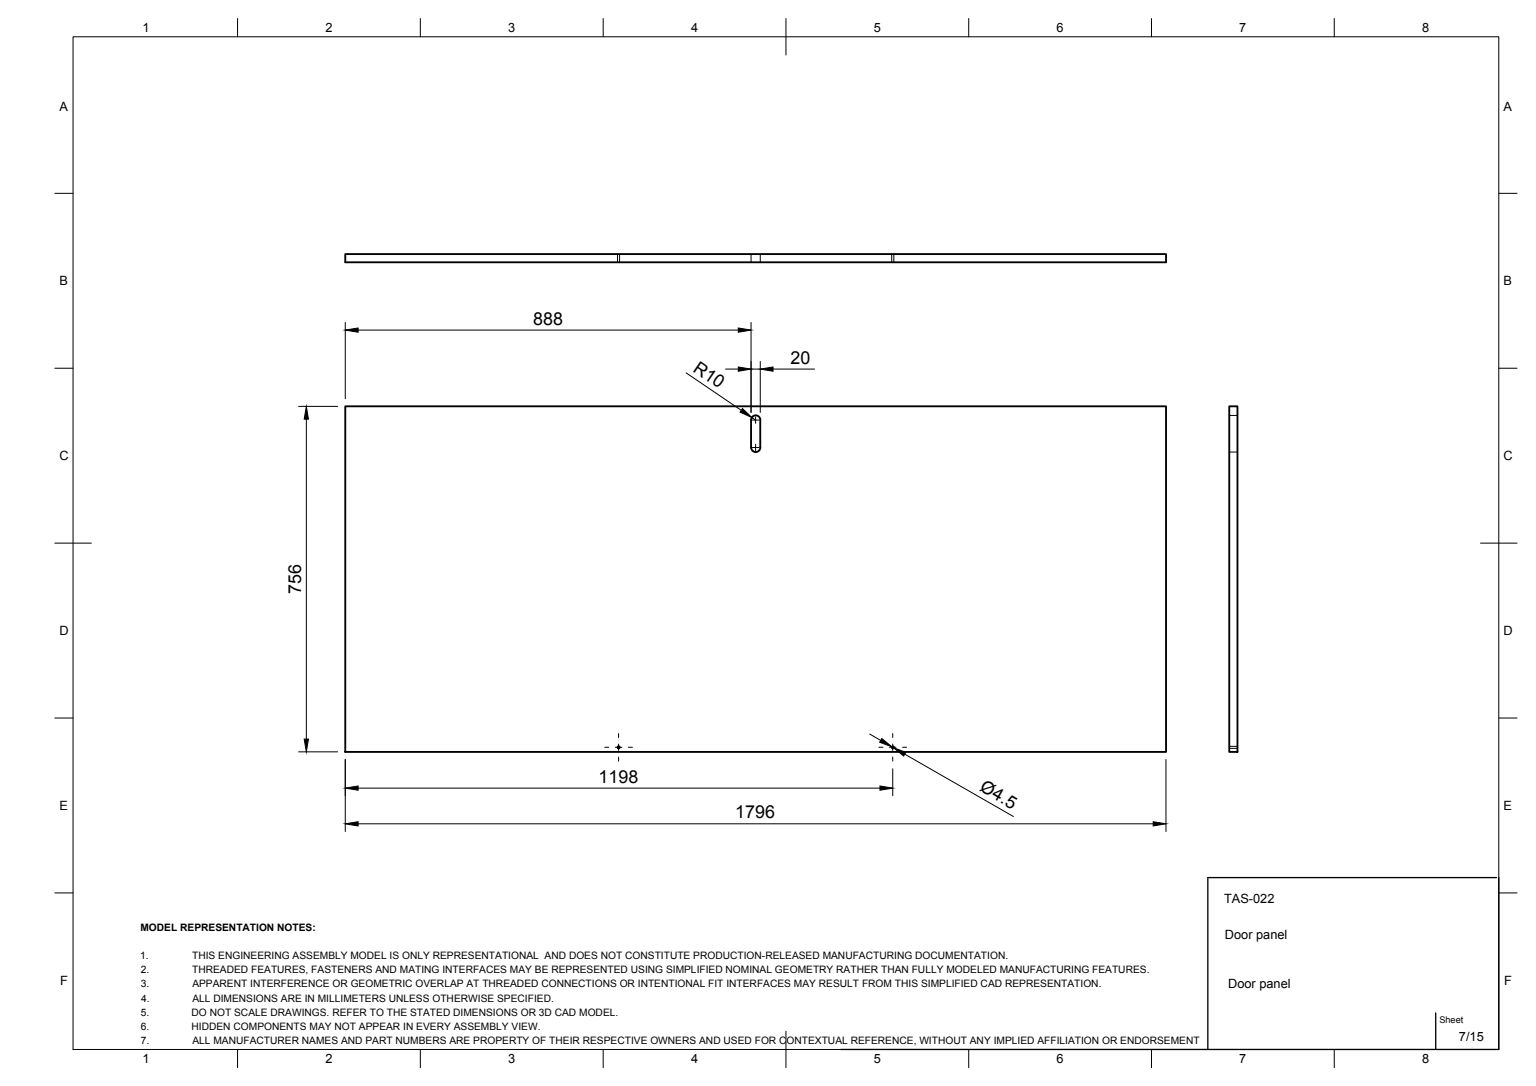
ISO-10303-21;
HEADER;
/* Generated by software containing ST-Developer
 * from STEP Tools, Inc. (www.steptools.com) 
 */

FILE_DESCRIPTION(
/* description */ (''),
/* implementation_level */ '2;1');

FILE_NAME(
/* name */ 'Door panel.step',
/* time_stamp */ '2026-11-15T21:02:08-08:00',
/* author */ (''),
/* organization */ (''),
/* preprocessor_version */ 'ST-DEVELOPER v20.2',
/* originating_system */ 'Autodesk Translation Framework v15.17.0.0',
/* authorisation */ '');

FILE_SCHEMA (('AUTOMOTIVE_DESIGN { 1 0 10303 214 3 1 1 }'));
ENDSEC;

DATA;
#10=MECHANICAL_DESIGN_GEOMETRIC_PRESENTATION_REPRESENTATION('',(#603),#31566);
#381=FACE_BOUND('',#914,.T.);
#382=FACE_BOUND('',#915,.T.);
#383=FACE_BOUND('',#916,.T.);
#384=FACE_BOUND('',#919,.T.);
#385=FACE_BOUND('',#920,.T.);
#386=FACE_BOUND('',#921,.T.);
#417=CIRCLE('',#5907,1.);
#418=CIRCLE('',#5908,1.);
#419=CIRCLE('',#5911,1.);
#420=CIRCLE('',#5912,1.);
#421=CIRCLE('',#5914,0.225);
#422=CIRCLE('',#5915,0.225);
#423=CIRCLE('',#5917,0.225);
#424=CIRCLE('',#5918,0.225);
#490=CYLINDRICAL_SURFACE('',#5906,1.);
#491=CYLINDRICAL_SURFACE('',#5910,1.);
#492=CYLINDRICAL_SURFACE('',#5913,0.225);
#493=CYLINDRICAL_SURFACE('',#5916,0.225);
#573=SHAPE_REPRESENTATION_RELATIONSHIP('SRR','None',#31637,#588);
#588=ADVANCED_BREP_SHAPE_REPRESENTATION('',(#618),#31552);
#603=STYLED_ITEM('',(#31721),#618);
#618=MANIFOLD_SOLID_BREP('Body1',#5716);
#638=FACE_OUTER_BOUND('',#907,.T.);
#639=FACE_OUTER_BOUND('',#908,.T.);
#640=FACE_OUTER_BOUND('',#909,.T.);
#641=FACE_OUTER_BOUND('',#910,.T.);
#642=FACE_OUTER_BOUND('',#911,.T.);
#643=FACE_OUTER_BOUND('',#912,.T.);
#644=FACE_OUTER_BOUND('',#913,.T.);
#645=FACE_OUTER_BOUND('',#917,.T.);
#646=FACE_OUTER_BOUND('',#918,.T.);
#647=FACE_OUTER_BOUND('',#922,.T.);
#648=FACE_OUTER_BOUND('',#923,.T.);
#649=FACE_OUTER_BOUND('',#924,.T.);
#907=EDGE_LOOP('',(#3651,#3652,#3653,#3654));
#908=EDGE_LOOP('',(#3655,#3656,#3657,#3658));
#909=EDGE_LOOP('',(#3659,#3660,#3661,#3662));
#910=EDGE_LOOP('',(#3663,#3664,#3665,#3666));
#911=EDGE_LOOP('',(#3667,#3668,#3669,#3670));
#912=EDGE_LOOP('',(#3671,#3672,#3673,#3674));
#913=EDGE_LOOP('',(#3675,#3676,#3677,#3678));
#914=EDGE_LOOP('',(#3679,#3680,#3681,#3682));
#915=EDGE_LOOP('',(#3683));
#916=EDGE_LOOP('',(#3684));
#917=EDGE_LOOP('',(#3685,#3686,#3687,#3688));
#918=EDGE_LOOP('',(#3689,#3690,#3691,#3692));
#919=EDGE_LOOP('',(#3693,#3694,#3695,#3696));
#920=EDGE_LOOP('',(#3697));
#921=EDGE_LOOP('',(#3698));
#922=EDGE_LOOP('',(#3699,#3700,#3701,#3702));
#923=EDGE_LOOP('',(#3703,#3704,#3705,#3706));
#924=EDGE_LOOP('',(#3707,#3708,#3709,#3710));
#1218=LINE('',#7593,#1725);
#1219=LINE('',#7595,#1726);
#1220=LINE('',#7597,#1727);
#1221=LINE('',#7598,#1728);
#1222=LINE('',#7603,#1729);
#1223=LINE('',#7607,#1730);
#1224=LINE('',#7609,#1731);
#1225=LINE('',#7610,#1732);
#1226=LINE('',#7618,#1733);
#1227=LINE('',#7624,#1734);
#1228=LINE('',#7629,#1735);
#1229=LINE('',#7631,#1736);
#1230=LINE('',#7633,#1737);
#1231=LINE('',#7634,#1738);
#1232=LINE('',#7637,#1739);
#1233=LINE('',#7639,#1740);
#1234=LINE('',#7640,#1741);
#1235=LINE('',#7643,#1742);
#1236=LINE('',#7645,#1743);
#1237=LINE('',#7646,#1744);
#1238=LINE('',#7648,#1745);
#1239=LINE('',#7649,#1746);
#1725=VECTOR('',#6314,1.);
#1726=VECTOR('',#6315,1.);
#1727=VECTOR('',#6316,1.);
#1728=VECTOR('',#6317,1.);
#1729=VECTOR('',#6322,1.);
#1730=VECTOR('',#6327,1.);
#1731=VECTOR('',#6328,1.);
#1732=VECTOR('',#6329,1.);
#1733=VECTOR('',#6340,0.225);
#1734=VECTOR('',#6347,0.225);
#1735=VECTOR('',#6352,1.);
#1736=VECTOR('',#6353,1.);
#1737=VECTOR('',#6354,1.);
#1738=VECTOR('',#6355,1.);
#1739=VECTOR('',#6358,1.);
#1740=VECTOR('',#6359,1.);
#1741=VECTOR('',#6360,1.);
#1742=VECTOR('',#6363,1.);
#1743=VECTOR('',#6364,1.);
#1744=VECTOR('',#6365,1.);
#1745=VECTOR('',#6368,1.);
#1746=VECTOR('',#6369,1.);
#2228=VERTEX_POINT('',#7591);
#2229=VERTEX_POINT('',#7592);
#2230=VERTEX_POINT('',#7594);
#2231=VERTEX_POINT('',#7596);
#2232=VERTEX_POINT('',#7600);
#2233=VERTEX_POINT('',#7602);
#2234=VERTEX_POINT('',#7606);
#2235=VERTEX_POINT('',#7608);
#2236=VERTEX_POINT('',#7615);
#2237=VERTEX_POINT('',#7617);
#2238=VERTEX_POINT('',#7621);
#2239=VERTEX_POINT('',#7623);
#2240=VERTEX_POINT('',#7627);
#2241=VERTEX_POINT('',#7628);
#2242=VERTEX_POINT('',#7630);
#2243=VERTEX_POINT('',#7632);
#2244=VERTEX_POINT('',#7636);
#2245=VERTEX_POINT('',#7638);
#2246=VERTEX_POINT('',#7642);
#2247=VERTEX_POINT('',#7644);
#2821=EDGE_CURVE('',#2228,#2229,#1218,.T.);
#2822=EDGE_CURVE('',#2228,#2230,#1219,.T.);
#2823=EDGE_CURVE('',#2231,#2230,#1220,.T.);
#2824=EDGE_CURVE('',#2229,#2231,#1221,.T.);
#2825=EDGE_CURVE('',#2232,#2228,#417,.T.);
#2826=EDGE_CURVE('',#2232,#2233,#1222,.T.);
#2827=EDGE_CURVE('',#2230,#2233,#418,.T.);
#2828=EDGE_CURVE('',#2234,#2232,#1223,.T.);
#2829=EDGE_CURVE('',#2234,#2235,#1224,.T.);
#2830=EDGE_CURVE('',#2233,#2235,#1225,.T.);
#2831=EDGE_CURVE('',#2229,#2234,#419,.T.);
#2832=EDGE_CURVE('',#2235,#2231,#420,.T.);
#2833=EDGE_CURVE('',#2236,#2236,#421,.T.);
#2834=EDGE_CURVE('',#2236,#2237,#1226,.T.);
#2835=EDGE_CURVE('',#2237,#2237,#422,.T.);
#2836=EDGE_CURVE('',#2238,#2238,#423,.T.);
#2837=EDGE_CURVE('',#2238,#2239,#1227,.T.);
#2838=EDGE_CURVE('',#2239,#2239,#424,.T.);
#2839=EDGE_CURVE('',#2240,#2241,#1228,.T.);
#2840=EDGE_CURVE('',#2241,#2242,#1229,.T.);
#2841=EDGE_CURVE('',#2243,#2242,#1230,.T.);
#2842=EDGE_CURVE('',#2240,#2243,#1231,.T.);
#2843=EDGE_CURVE('',#2244,#2240,#1232,.T.);
#2844=EDGE_CURVE('',#2245,#2243,#1233,.T.);
#2845=EDGE_CURVE('',#2244,#2245,#1234,.T.);
#2846=EDGE_CURVE('',#2246,#2244,#1235,.T.);
#2847=EDGE_CURVE('',#2247,#2245,#1236,.T.);
#2848=EDGE_CURVE('',#2246,#2247,#1237,.T.);
#2849=EDGE_CURVE('',#2241,#2246,#1238,.T.);
#2850=EDGE_CURVE('',#2242,#2247,#1239,.T.);
#3651=ORIENTED_EDGE('',*,*,#2821,.F.);
#3652=ORIENTED_EDGE('',*,*,#2822,.T.);
#3653=ORIENTED_EDGE('',*,*,#2823,.F.);
#3654=ORIENTED_EDGE('',*,*,#2824,.F.);
#3655=ORIENTED_EDGE('',*,*,#2825,.F.);
#3656=ORIENTED_EDGE('',*,*,#2826,.T.);
#3657=ORIENTED_EDGE('',*,*,#2827,.F.);
#3658=ORIENTED_EDGE('',*,*,#2822,.F.);
#3659=ORIENTED_EDGE('',*,*,#2828,.F.);
#3660=ORIENTED_EDGE('',*,*,#2829,.T.);
#3661=ORIENTED_EDGE('',*,*,#2830,.F.);
#3662=ORIENTED_EDGE('',*,*,#2826,.F.);
#3663=ORIENTED_EDGE('',*,*,#2831,.F.);
#3664=ORIENTED_EDGE('',*,*,#2824,.T.);
#3665=ORIENTED_EDGE('',*,*,#2832,.F.);
#3666=ORIENTED_EDGE('',*,*,#2829,.F.);
#3667=ORIENTED_EDGE('',*,*,#2833,.F.);
#3668=ORIENTED_EDGE('',*,*,#2834,.T.);
#3669=ORIENTED_EDGE('',*,*,#2835,.F.);
#3670=ORIENTED_EDGE('',*,*,#2834,.F.);
#3671=ORIENTED_EDGE('',*,*,#2836,.F.);
#3672=ORIENTED_EDGE('',*,*,#2837,.T.);
#3673=ORIENTED_EDGE('',*,*,#2838,.F.);
#3674=ORIENTED_EDGE('',*,*,#2837,.F.);
#3675=ORIENTED_EDGE('',*,*,#2839,.T.);
#3676=ORIENTED_EDGE('',*,*,#2840,.T.);
#3677=ORIENTED_EDGE('',*,*,#2841,.F.);
#3678=ORIENTED_EDGE('',*,*,#2842,.F.);
#3679=ORIENTED_EDGE('',*,*,#2821,.T.);
#3680=ORIENTED_EDGE('',*,*,#2831,.T.);
#3681=ORIENTED_EDGE('',*,*,#2828,.T.);
#3682=ORIENTED_EDGE('',*,*,#2825,.T.);
#3683=ORIENTED_EDGE('',*,*,#2833,.T.);
#3684=ORIENTED_EDGE('',*,*,#2836,.T.);
#3685=ORIENTED_EDGE('',*,*,#2843,.T.);
#3686=ORIENTED_EDGE('',*,*,#2842,.T.);
#3687=ORIENTED_EDGE('',*,*,#2844,.F.);
#3688=ORIENTED_EDGE('',*,*,#2845,.F.);
#3689=ORIENTED_EDGE('',*,*,#2846,.T.);
#3690=ORIENTED_EDGE('',*,*,#2845,.T.);
#3691=ORIENTED_EDGE('',*,*,#2847,.F.);
#3692=ORIENTED_EDGE('',*,*,#2848,.F.);
#3693=ORIENTED_EDGE('',*,*,#2823,.T.);
#3694=ORIENTED_EDGE('',*,*,#2827,.T.);
#3695=ORIENTED_EDGE('',*,*,#2830,.T.);
#3696=ORIENTED_EDGE('',*,*,#2832,.T.);
#3697=ORIENTED_EDGE('',*,*,#2835,.T.);
#3698=ORIENTED_EDGE('',*,*,#2838,.T.);
#3699=ORIENTED_EDGE('',*,*,#2849,.T.);
#3700=ORIENTED_EDGE('',*,*,#2848,.T.);
#3701=ORIENTED_EDGE('',*,*,#2850,.F.);
#3702=ORIENTED_EDGE('',*,*,#2840,.F.);
#3703=ORIENTED_EDGE('',*,*,#2850,.T.);
#3704=ORIENTED_EDGE('',*,*,#2847,.T.);
#3705=ORIENTED_EDGE('',*,*,#2844,.T.);
#3706=ORIENTED_EDGE('',*,*,#2841,.T.);
#3707=ORIENTED_EDGE('',*,*,#2849,.F.);
#3708=ORIENTED_EDGE('',*,*,#2839,.F.);
#3709=ORIENTED_EDGE('',*,*,#2843,.F.);
#3710=ORIENTED_EDGE('',*,*,#2846,.F.);
#5269=PLANE('',#5905);
#5270=PLANE('',#5909);
#5271=PLANE('',#5919);
#5272=PLANE('',#5920);
#5273=PLANE('',#5921);
#5274=PLANE('',#5922);
#5275=PLANE('',#5923);
#5276=PLANE('',#5924);
#5452=ADVANCED_FACE('',(#638),#5269,.F.);
#5453=ADVANCED_FACE('',(#639),#490,.F.);
#5454=ADVANCED_FACE('',(#640),#5270,.F.);
#5455=ADVANCED_FACE('',(#641),#491,.F.);
#5456=ADVANCED_FACE('',(#642),#492,.F.);
#5457=ADVANCED_FACE('',(#643),#493,.F.);
#5458=ADVANCED_FACE('',(#644,#381,#382,#383),#5271,.T.);
#5459=ADVANCED_FACE('',(#645),#5272,.T.);
#5460=ADVANCED_FACE('',(#646,#384,#385,#386),#5273,.T.);
#5461=ADVANCED_FACE('',(#647),#5274,.T.);
#5462=ADVANCED_FACE('',(#648),#5275,.T.);
#5463=ADVANCED_FACE('',(#649),#5276,.F.);
#5716=CLOSED_SHELL('',(#5452,#5453,#5454,#5455,#5456,#5457,#5458,#5459,
#5460,#5461,#5462,#5463));
#5904=AXIS2_PLACEMENT_3D('',#7589,#6310,#6311);
#5905=AXIS2_PLACEMENT_3D('',#7590,#6312,#6313);
#5906=AXIS2_PLACEMENT_3D('',#7599,#6318,#6319);
#5907=AXIS2_PLACEMENT_3D('',#7601,#6320,#6321);
#5908=AXIS2_PLACEMENT_3D('',#7604,#6323,#6324);
#5909=AXIS2_PLACEMENT_3D('',#7605,#6325,#6326);
#5910=AXIS2_PLACEMENT_3D('',#7611,#6330,#6331);
#5911=AXIS2_PLACEMENT_3D('',#7612,#6332,#6333);
#5912=AXIS2_PLACEMENT_3D('',#7613,#6334,#6335);
#5913=AXIS2_PLACEMENT_3D('',#7614,#6336,#6337);
#5914=AXIS2_PLACEMENT_3D('',#7616,#6338,#6339);
#5915=AXIS2_PLACEMENT_3D('',#7619,#6341,#6342);
#5916=AXIS2_PLACEMENT_3D('',#7620,#6343,#6344);
#5917=AXIS2_PLACEMENT_3D('',#7622,#6345,#6346);
#5918=AXIS2_PLACEMENT_3D('',#7625,#6348,#6349);
#5919=AXIS2_PLACEMENT_3D('',#7626,#6350,#6351);
#5920=AXIS2_PLACEMENT_3D('',#7635,#6356,#6357);
#5921=AXIS2_PLACEMENT_3D('',#7641,#6361,#6362);
#5922=AXIS2_PLACEMENT_3D('',#7647,#6366,#6367);
#5923=AXIS2_PLACEMENT_3D('',#7650,#6370,#6371);
#5924=AXIS2_PLACEMENT_3D('',#7651,#6372,#6373);
#6310=DIRECTION('axis',(0.,0.,1.));
#6311=DIRECTION('refdir',(1.,0.,0.));
#6312=DIRECTION('center_axis',(0.,0.,-1.));
#6313=DIRECTION('ref_axis',(1.,0.,0.));
#6314=DIRECTION('',(1.,0.,0.));
#6315=DIRECTION('',(0.,-1.,0.));
#6316=DIRECTION('',(-1.,0.,0.));
#6317=DIRECTION('',(0.,-1.,0.));
#6318=DIRECTION('center_axis',(0.,-1.,0.));
#6319=DIRECTION('ref_axis',(0.,0.,-1.));
#6320=DIRECTION('center_axis',(0.,-1.,0.));
#6321=DIRECTION('ref_axis',(0.,0.,-1.));
#6322=DIRECTION('',(0.,-1.,0.));
#6323=DIRECTION('center_axis',(0.,1.,0.));
#6324=DIRECTION('ref_axis',(0.,0.,-1.));
#6325=DIRECTION('center_axis',(0.,0.,1.));
#6326=DIRECTION('ref_axis',(-1.,0.,0.));
#6327=DIRECTION('',(-1.,0.,0.));
#6328=DIRECTION('',(0.,-1.,0.));
#6329=DIRECTION('',(1.,0.,0.));
#6330=DIRECTION('center_axis',(0.,-1.,0.));
#6331=DIRECTION('ref_axis',(0.,0.,1.));
#6332=DIRECTION('center_axis',(0.,-1.,0.));
#6333=DIRECTION('ref_axis',(0.,0.,1.));
#6334=DIRECTION('center_axis',(0.,1.,0.));
#6335=DIRECTION('ref_axis',(0.,0.,1.));
#6336=DIRECTION('center_axis',(0.,-1.,0.));
#6337=DIRECTION('ref_axis',(1.,0.,0.));
#6338=DIRECTION('center_axis',(0.,-1.,0.));
#6339=DIRECTION('ref_axis',(1.,0.,0.));
#6340=DIRECTION('',(0.,-1.,0.));
#6341=DIRECTION('center_axis',(0.,1.,0.));
#6342=DIRECTION('ref_axis',(1.,0.,0.));
#6343=DIRECTION('center_axis',(0.,-1.,0.));
#6344=DIRECTION('ref_axis',(1.,0.,0.));
#6345=DIRECTION('center_axis',(0.,-1.,0.));
#6346=DIRECTION('ref_axis',(1.,0.,0.));
#6347=DIRECTION('',(0.,-1.,0.));
#6348=DIRECTION('center_axis',(0.,1.,0.));
#6349=DIRECTION('ref_axis',(1.,0.,0.));
#6350=DIRECTION('center_axis',(0.,1.,0.));
#6351=DIRECTION('ref_axis',(-1.,0.,0.));
#6352=DIRECTION('',(-1.,0.,0.));
#6353=DIRECTION('',(0.,0.,1.));
#6354=DIRECTION('',(-1.,0.,0.));
#6355=DIRECTION('',(0.,0.,1.));
#6356=DIRECTION('center_axis',(1.,0.,0.));
#6357=DIRECTION('ref_axis',(0.,1.,0.));
#6358=DIRECTION('',(0.,1.,0.));
#6359=DIRECTION('',(0.,1.,0.));
#6360=DIRECTION('',(0.,0.,1.));
#6361=DIRECTION('center_axis',(0.,-1.,0.));
#6362=DIRECTION('ref_axis',(1.,0.,0.));
#6363=DIRECTION('',(1.,0.,0.));
#6364=DIRECTION('',(1.,0.,0.));
#6365=DIRECTION('',(0.,0.,1.));
#6366=DIRECTION('center_axis',(-1.,0.,0.));
#6367=DIRECTION('ref_axis',(0.,-1.,0.));
#6368=DIRECTION('',(0.,-1.,0.));
#6369=DIRECTION('',(0.,-1.,0.));
#6370=DIRECTION('center_axis',(0.,0.,1.));
#6371=DIRECTION('ref_axis',(1.,0.,0.));
#6372=DIRECTION('center_axis',(0.,0.,1.));
#6373=DIRECTION('ref_axis',(1.,0.,0.));
#7589=CARTESIAN_POINT('',(0.,0.,0.));
#7590=CARTESIAN_POINT('Origin',(69.,-0.2,89.));
#7591=CARTESIAN_POINT('',(69.,-0.2,89.));
#7592=CARTESIAN_POINT('',(75.,-0.2,89.));
#7593=CARTESIAN_POINT('',(73.5,-0.2,89.));
#7594=CARTESIAN_POINT('',(69.,-2.,89.));
#7595=CARTESIAN_POINT('',(69.,-0.2,89.));
#7596=CARTESIAN_POINT('',(75.,-2.,89.));
#7597=CARTESIAN_POINT('',(35.7,-2.,89.));
#7598=CARTESIAN_POINT('',(75.,-0.2,89.));
#7599=CARTESIAN_POINT('Origin',(69.,-0.2,90.));
#7600=CARTESIAN_POINT('',(69.,-0.2,91.));
#7601=CARTESIAN_POINT('Origin',(69.,-0.2,90.));
#7602=CARTESIAN_POINT('',(69.,-2.,91.));
#7603=CARTESIAN_POINT('',(69.,-0.2,91.));
#7604=CARTESIAN_POINT('Origin',(69.,-2.,90.));
#7605=CARTESIAN_POINT('Origin',(75.,-0.2,91.));
#7606=CARTESIAN_POINT('',(75.,-0.2,91.));
#7607=CARTESIAN_POINT('',(76.5,-0.2,91.));
#7608=CARTESIAN_POINT('',(75.,-2.,91.));
#7609=CARTESIAN_POINT('',(75.,-0.2,91.));
#7610=CARTESIAN_POINT('',(38.7,-2.,91.));
#7611=CARTESIAN_POINT('Origin',(75.,-0.2,90.));
#7612=CARTESIAN_POINT('Origin',(75.,-0.2,90.));
#7613=CARTESIAN_POINT('Origin',(75.,-2.,90.));
#7614=CARTESIAN_POINT('Origin',(3.4,-0.2,60.));
#7615=CARTESIAN_POINT('',(3.175,-0.2,60.));
#7616=CARTESIAN_POINT('Origin',(3.4,-0.2,60.));
#7617=CARTESIAN_POINT('',(3.175,-2.,60.));
#7618=CARTESIAN_POINT('',(3.175,-0.2,60.));
#7619=CARTESIAN_POINT('Origin',(3.4,-2.,60.));
#7620=CARTESIAN_POINT('Origin',(3.4,-0.2,120.));
#7621=CARTESIAN_POINT('',(3.175,-0.2,120.));
#7622=CARTESIAN_POINT('Origin',(3.4,-0.2,120.));
#7623=CARTESIAN_POINT('',(3.175,-2.,120.));
#7624=CARTESIAN_POINT('',(3.175,-0.2,120.));
#7625=CARTESIAN_POINT('Origin',(3.4,-2.,120.));
#7626=CARTESIAN_POINT('Origin',(78.,-0.2,0.2));
#7627=CARTESIAN_POINT('',(78.,-0.2,0.2));
#7628=CARTESIAN_POINT('',(2.4,-0.2,0.2));
#7629=CARTESIAN_POINT('',(78.,-0.2,0.2));
#7630=CARTESIAN_POINT('',(2.4,-0.2,179.8));
#7631=CARTESIAN_POINT('',(2.4,-0.2,0.2));
#7632=CARTESIAN_POINT('',(78.,-0.2,179.8));
#7633=CARTESIAN_POINT('',(78.,-0.2,179.8));
#7634=CARTESIAN_POINT('',(78.,-0.2,0.2));
#7635=CARTESIAN_POINT('Origin',(78.,-2.,0.2));
#7636=CARTESIAN_POINT('',(78.,-2.,0.2));
#7637=CARTESIAN_POINT('',(78.,-2.,0.2));
#7638=CARTESIAN_POINT('',(78.,-2.,179.8));
#7639=CARTESIAN_POINT('',(78.,-2.,179.8));
#7640=CARTESIAN_POINT('',(78.,-2.,0.2));
#7641=CARTESIAN_POINT('Origin',(2.4,-2.,0.2));
#7642=CARTESIAN_POINT('',(2.4,-2.,0.2));
#7643=CARTESIAN_POINT('',(2.4,-2.,0.2));
#7644=CARTESIAN_POINT('',(2.4,-2.,179.8));
#7645=CARTESIAN_POINT('',(2.4,-2.,179.8));
#7646=CARTESIAN_POINT('',(2.4,-2.,0.2));
#7647=CARTESIAN_POINT('Origin',(2.4,-0.2,0.2));
#7648=CARTESIAN_POINT('',(2.4,-0.2,0.2));
#7649=CARTESIAN_POINT('',(2.4,-0.2,179.8));
#7650=CARTESIAN_POINT('Origin',(40.2,-1.1,179.8));
#7651=CARTESIAN_POINT('Origin',(40.2,-1.1,0.2));
#31535=UNCERTAINTY_MEASURE_WITH_UNIT(LENGTH_MEASURE(0.001),#31567,
'DISTANCE_ACCURACY_VALUE',
'Maximum model space distance between geometric entities at asserted c
onnectivities');
#31549=UNCERTAINTY_MEASURE_WITH_UNIT(LENGTH_MEASURE(0.001),#31567,
'DISTANCE_ACCURACY_VALUE',
'Maximum model space distance between geometric entities at asserted c
onnectivities');
#31552=(
GEOMETRIC_REPRESENTATION_CONTEXT(3)
GLOBAL_UNCERTAINTY_ASSIGNED_CONTEXT((#31535))
GLOBAL_UNIT_ASSIGNED_CONTEXT((#31567,#31569,#31570))
REPRESENTATION_CONTEXT('','3D')
);
#31566=(
GEOMETRIC_REPRESENTATION_CONTEXT(3)
GLOBAL_UNCERTAINTY_ASSIGNED_CONTEXT((#31549))
GLOBAL_UNIT_ASSIGNED_CONTEXT((#31567,#31569,#31570))
REPRESENTATION_CONTEXT('','3D')
);
#31567=(
LENGTH_UNIT()
NAMED_UNIT(*)
SI_UNIT(.CENTI.,.METRE.)
);
#31569=(
NAMED_UNIT(*)
PLANE_ANGLE_UNIT()
SI_UNIT($,.RADIAN.)
);
#31570=(
NAMED_UNIT(*)
SI_UNIT($,.STERADIAN.)
SOLID_ANGLE_UNIT()
);
#31573=SHAPE_DEFINITION_REPRESENTATION(#31589,#31637);
#31589=PRODUCT_DEFINITION_SHAPE('',$,#31654);
#31637=SHAPE_REPRESENTATION('',(#5904),#31552);
#31651=PRODUCT_DEFINITION_CONTEXT('part definition',#31701,'design');
#31654=PRODUCT_DEFINITION('Door panel','Door panel',#31670,#31651);
#31670=PRODUCT_DEFINITION_FORMATION('',$,#31705);
#31701=APPLICATION_CONTEXT(
'Core Data for Automotive Mechanical Design Process');
#31702=PRODUCT_CONTEXT('part definition',#31701,'mechanical');
#31705=PRODUCT('Door panel','Door panel','Door panel',(#31702));
#31721=PRESENTATION_STYLE_ASSIGNMENT((#31728));
#31728=SURFACE_STYLE_USAGE(.BOTH.,#31735);
#31735=SURFACE_SIDE_STYLE('',(#31742));
#31742=SURFACE_STYLE_FILL_AREA(#31749);
#31749=FILL_AREA_STYLE('Opaque(70,153,204)',(#31756));
#31756=FILL_AREA_STYLE_COLOUR('Opaque(70,153,204)',#31763);
#31763=COLOUR_RGB('Opaque(70,153,204)',0.274509803921569,0.6,0.8);
ENDSEC;
END-ISO-10303-21;
